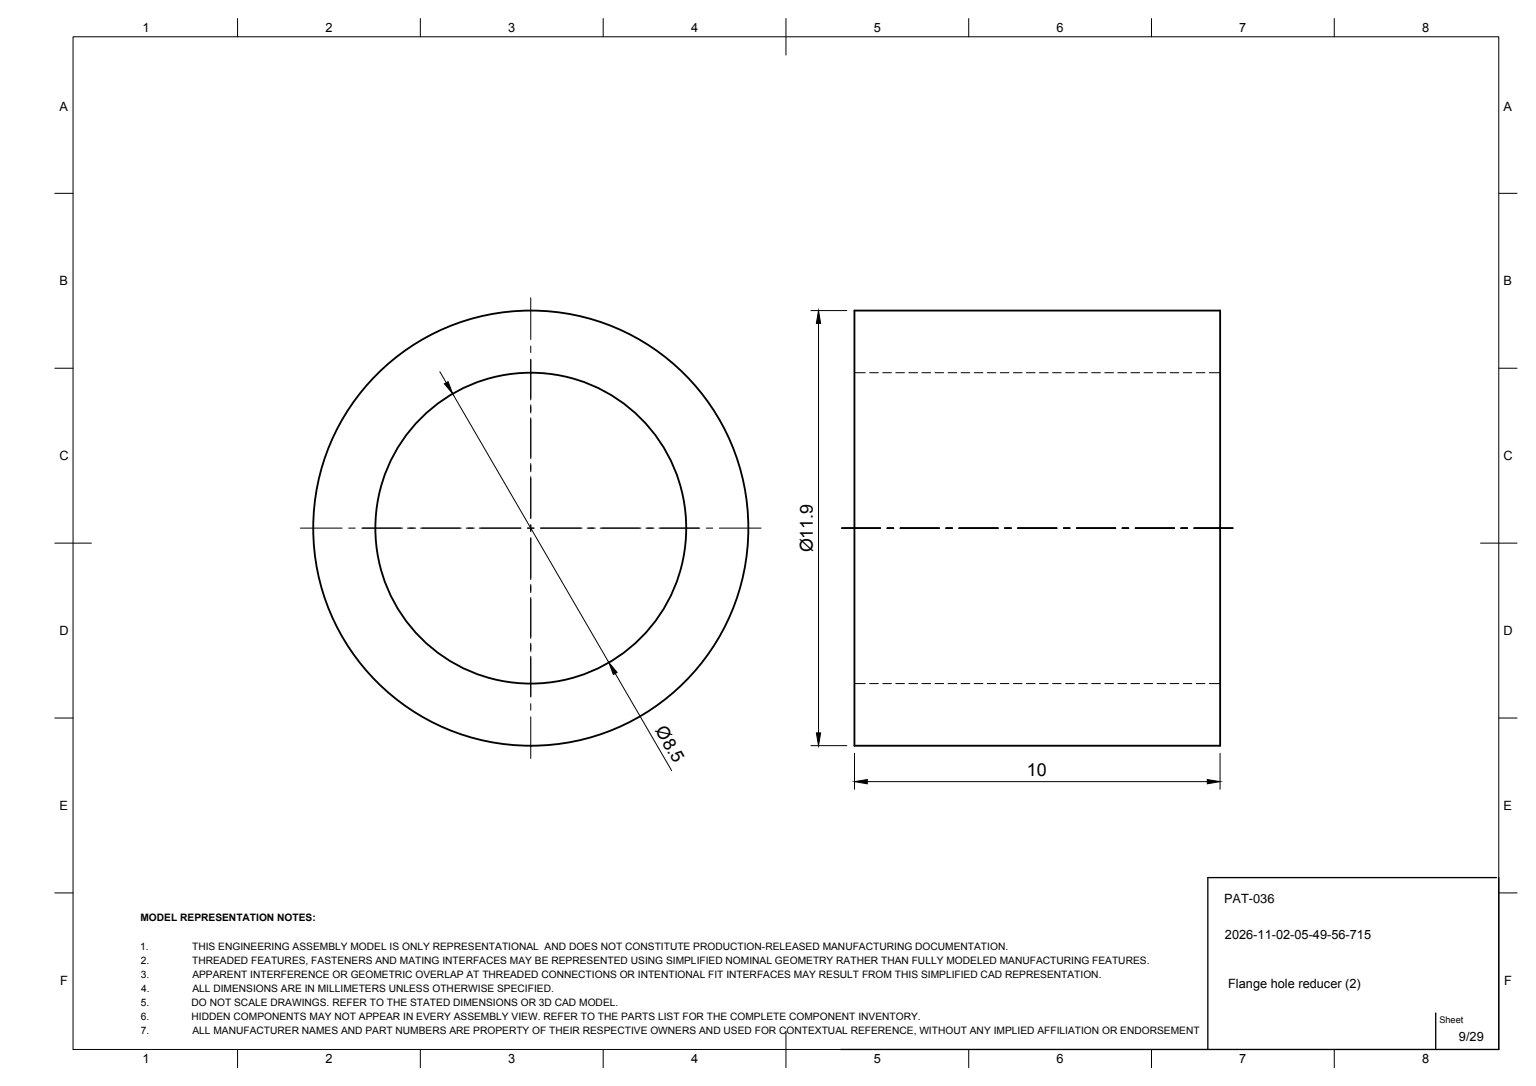
ISO-10303-21;
HEADER;
/* Generated by software containing ST-Developer
 * from STEP Tools, Inc. (www.steptools.com) 
 */

FILE_DESCRIPTION(
/* description */ ('Flange-mounted spindle'),
/* implementation_level */ '2;1');

FILE_NAME(
/* name */ 'Flange hole reducer (2).step',
/* time_stamp */ '2026-10-27T10:49:51-07:00',
/* author */ (''),
/* organization */ (''),
/* preprocessor_version */ 'ST-DEVELOPER v20.2',
/* originating_system */ 'Autodesk Translation Framework v15.17.0.0',
/* authorisation */ '');

FILE_SCHEMA (('AUTOMOTIVE_DESIGN { 1 0 10303 214 3 1 1 }'));
ENDSEC;

DATA;
#10=MECHANICAL_DESIGN_GEOMETRIC_PRESENTATION_REPRESENTATION('',(#342),#11764);
#288=SHAPE_REPRESENTATION_RELATIONSHIP('SRR','None',#11884,#315);
#315=ADVANCED_BREP_SHAPE_REPRESENTATION('',(#370),#11739);
#342=STYLED_ITEM('',(#12113),#370);
#370=MANIFOLD_SOLID_BREP('Body1',#6134);
#413=FACE_BOUND('',#1075,.T.);
#414=FACE_BOUND('',#1077,.T.);
#524=PLANE('',#6529);
#525=PLANE('',#6530);
#705=FACE_OUTER_BOUND('',#1072,.T.);
#706=FACE_OUTER_BOUND('',#1073,.T.);
#707=FACE_OUTER_BOUND('',#1074,.T.);
#708=FACE_OUTER_BOUND('',#1076,.T.);
#1072=EDGE_LOOP('',(#4143,#4144,#4145,#4146));
#1073=EDGE_LOOP('',(#4147,#4148,#4149,#4150));
#1074=EDGE_LOOP('',(#4151));
#1075=EDGE_LOOP('',(#4152));
#1076=EDGE_LOOP('',(#4153));
#1077=EDGE_LOOP('',(#4154));
#1522=LINE('',#9285,#1944);
#1523=LINE('',#9291,#1945);
#1944=VECTOR('',#7383,0.425);
#1945=VECTOR('',#7390,0.595);
#2349=CIRCLE('',#6524,0.425);
#2350=CIRCLE('',#6525,0.425);
#2351=CIRCLE('',#6527,0.595);
#2352=CIRCLE('',#6528,0.595);
#2695=VERTEX_POINT('',#9282);
#2696=VERTEX_POINT('',#9284);
#2697=VERTEX_POINT('',#9288);
#2698=VERTEX_POINT('',#9290);
#3264=EDGE_CURVE('',#2695,#2695,#2349,.T.);
#3265=EDGE_CURVE('',#2695,#2696,#1522,.T.);
#3266=EDGE_CURVE('',#2696,#2696,#2350,.T.);
#3267=EDGE_CURVE('',#2697,#2697,#2351,.T.);
#3268=EDGE_CURVE('',#2697,#2698,#1523,.T.);
#3269=EDGE_CURVE('',#2698,#2698,#2352,.T.);
#4143=ORIENTED_EDGE('',*,*,#3264,.F.);
#4144=ORIENTED_EDGE('',*,*,#3265,.T.);
#4145=ORIENTED_EDGE('',*,*,#3266,.T.);
#4146=ORIENTED_EDGE('',*,*,#3265,.F.);
#4147=ORIENTED_EDGE('',*,*,#3267,.F.);
#4148=ORIENTED_EDGE('',*,*,#3268,.T.);
#4149=ORIENTED_EDGE('',*,*,#3269,.T.);
#4150=ORIENTED_EDGE('',*,*,#3268,.F.);
#4151=ORIENTED_EDGE('',*,*,#3267,.T.);
#4152=ORIENTED_EDGE('',*,*,#3264,.T.);
#4153=ORIENTED_EDGE('',*,*,#3269,.F.);
#4154=ORIENTED_EDGE('',*,*,#3266,.F.);
#5638=CYLINDRICAL_SURFACE('',#6523,0.425);
#5639=CYLINDRICAL_SURFACE('',#6526,0.595);
#5816=ADVANCED_FACE('',(#705),#5638,.F.);
#5817=ADVANCED_FACE('',(#706),#5639,.T.);
#5818=ADVANCED_FACE('',(#707,#413),#524,.T.);
#5819=ADVANCED_FACE('',(#708,#414),#525,.F.);
#6134=CLOSED_SHELL('',(#5816,#5817,#5818,#5819));
#6522=AXIS2_PLACEMENT_3D('',#9280,#7377,#7378);
#6523=AXIS2_PLACEMENT_3D('',#9281,#7379,#7380);
#6524=AXIS2_PLACEMENT_3D('',#9283,#7381,#7382);
#6525=AXIS2_PLACEMENT_3D('',#9286,#7384,#7385);
#6526=AXIS2_PLACEMENT_3D('',#9287,#7386,#7387);
#6527=AXIS2_PLACEMENT_3D('',#9289,#7388,#7389);
#6528=AXIS2_PLACEMENT_3D('',#9292,#7391,#7392);
#6529=AXIS2_PLACEMENT_3D('',#9293,#7393,#7394);
#6530=AXIS2_PLACEMENT_3D('',#9294,#7395,#7396);
#7377=DIRECTION('axis',(0.,0.,1.));
#7378=DIRECTION('refdir',(1.,0.,0.));
#7379=DIRECTION('center_axis',(0.,1.,0.));
#7380=DIRECTION('ref_axis',(1.,0.,0.));
#7381=DIRECTION('center_axis',(0.,-1.,0.));
#7382=DIRECTION('ref_axis',(1.,0.,0.));
#7383=DIRECTION('',(0.,-1.,0.));
#7384=DIRECTION('center_axis',(0.,-1.,0.));
#7385=DIRECTION('ref_axis',(1.,0.,0.));
#7386=DIRECTION('center_axis',(0.,1.,0.));
#7387=DIRECTION('ref_axis',(1.,0.,0.));
#7388=DIRECTION('center_axis',(0.,1.,0.));
#7389=DIRECTION('ref_axis',(1.,0.,0.));
#7390=DIRECTION('',(0.,-1.,0.));
#7391=DIRECTION('center_axis',(0.,1.,0.));
#7392=DIRECTION('ref_axis',(1.,0.,0.));
#7393=DIRECTION('center_axis',(0.,1.,0.));
#7394=DIRECTION('ref_axis',(1.,0.,0.));
#7395=DIRECTION('center_axis',(0.,1.,0.));
#7396=DIRECTION('ref_axis',(1.,0.,0.));
#9280=CARTESIAN_POINT('',(0.,0.,0.));
#9281=CARTESIAN_POINT('Origin',(3.2,-0.5,4.8));
#9282=CARTESIAN_POINT('',(2.775,0.5,4.8));
#9283=CARTESIAN_POINT('Origin',(3.2,0.5,4.8));
#9284=CARTESIAN_POINT('',(2.775,-0.5,4.8));
#9285=CARTESIAN_POINT('',(2.775,-0.5,4.8));
#9286=CARTESIAN_POINT('Origin',(3.2,-0.5,4.8));
#9287=CARTESIAN_POINT('Origin',(3.2,-0.5,4.8));
#9288=CARTESIAN_POINT('',(2.605,0.5,4.8));
#9289=CARTESIAN_POINT('Origin',(3.2,0.5,4.8));
#9290=CARTESIAN_POINT('',(2.605,-0.5,4.8));
#9291=CARTESIAN_POINT('',(2.605,-0.5,4.8));
#9292=CARTESIAN_POINT('Origin',(3.2,-0.5,4.8));
#9293=CARTESIAN_POINT('Origin',(3.2,0.5,4.8));
#9294=CARTESIAN_POINT('Origin',(3.2,-0.5,4.8));
#11707=UNCERTAINTY_MEASURE_WITH_UNIT(LENGTH_MEASURE(0.001),#11765,
'DISTANCE_ACCURACY_VALUE',
'Maximum model space distance between geometric entities at asserted c
onnectivities');
#11732=UNCERTAINTY_MEASURE_WITH_UNIT(LENGTH_MEASURE(0.001),#11765,
'DISTANCE_ACCURACY_VALUE',
'Maximum model space distance between geometric entities at asserted c
onnectivities');
#11739=(
GEOMETRIC_REPRESENTATION_CONTEXT(3)
GLOBAL_UNCERTAINTY_ASSIGNED_CONTEXT((#11707))
GLOBAL_UNIT_ASSIGNED_CONTEXT((#11765,#11767,#11768))
REPRESENTATION_CONTEXT('','3D')
);
#11764=(
GEOMETRIC_REPRESENTATION_CONTEXT(3)
GLOBAL_UNCERTAINTY_ASSIGNED_CONTEXT((#11732))
GLOBAL_UNIT_ASSIGNED_CONTEXT((#11765,#11767,#11768))
REPRESENTATION_CONTEXT('','3D')
);
#11765=(
LENGTH_UNIT()
NAMED_UNIT(*)
SI_UNIT(.CENTI.,.METRE.)
);
#11767=(
NAMED_UNIT(*)
PLANE_ANGLE_UNIT()
SI_UNIT($,.RADIAN.)
);
#11768=(
NAMED_UNIT(*)
SI_UNIT($,.STERADIAN.)
SOLID_ANGLE_UNIT()
);
#11775=SHAPE_DEFINITION_REPRESENTATION(#11806,#11884);
#11806=PRODUCT_DEFINITION_SHAPE('',$,#11916);
#11884=SHAPE_REPRESENTATION('',(#6522),#11739);
#11909=PRODUCT_DEFINITION_CONTEXT('part definition',#12004,'design');
#11916=PRODUCT_DEFINITION('Flange hole reducer (2)',
'Flange hole reducer (2)',#11947,#11909);
#11947=PRODUCT_DEFINITION_FORMATION('',$,#12012);
#12004=APPLICATION_CONTEXT(
'Core Data for Automotive Mechanical Design Process');
#12005=PRODUCT_CONTEXT('part definition',#12004,'mechanical');
#12012=PRODUCT('Flange hole reducer (2)','Flange hole reducer (2)',
'Flange hole reducer (2)',(#12005));
#12107=COLOUR_RGB('Off White',0.89,0.88,0.83);
#12108=FILL_AREA_STYLE_COLOUR('',#12107);
#12109=FILL_AREA_STYLE('',(#12108));
#12110=SURFACE_STYLE_FILL_AREA(#12109);
#12111=SURFACE_SIDE_STYLE('',(#12110));
#12112=SURFACE_STYLE_USAGE(.BOTH.,#12111);
#12113=PRESENTATION_STYLE_ASSIGNMENT((#12112));
ENDSEC;
END-ISO-10303-21;
